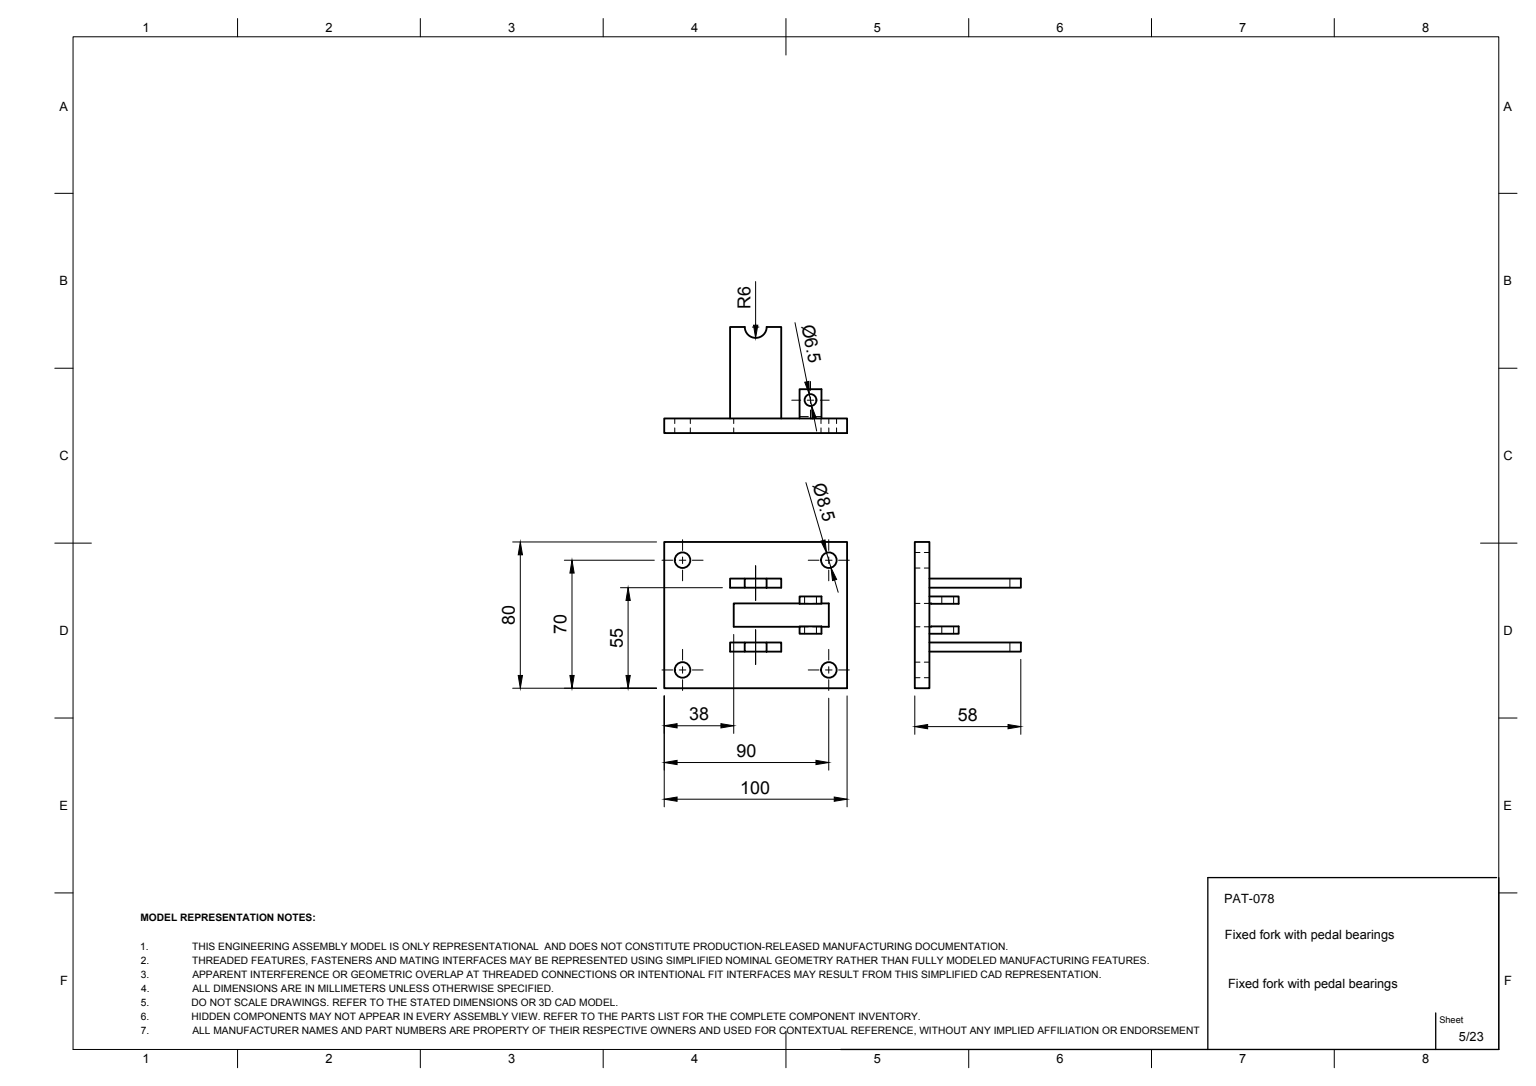
ISO-10303-21;
HEADER;
/* Generated by software containing ST-Developer
 * from STEP Tools, Inc. (www.steptools.com) 
 */

FILE_DESCRIPTION(
/* description */ ('Pedal-braked fixed caster'),
/* implementation_level */ '2;1');

FILE_NAME(
/* name */ 'Fixed fork with pedal bearings.step',
/* time_stamp */ '2026-10-28T03:26:52-07:00',
/* author */ (''),
/* organization */ (''),
/* preprocessor_version */ 'ST-DEVELOPER v20.2',
/* originating_system */ 'Autodesk Translation Framework v15.17.0.0',
/* authorisation */ '');

FILE_SCHEMA (('AUTOMOTIVE_DESIGN { 1 0 10303 214 3 1 1 }'));
ENDSEC;

DATA;
#10=MECHANICAL_DESIGN_GEOMETRIC_PRESENTATION_REPRESENTATION('',(#206),#5734);
#172=SHAPE_REPRESENTATION_RELATIONSHIP('SRR','None',#5810,#189);
#189=ADVANCED_BREP_SHAPE_REPRESENTATION('',(#230),#5714);
#206=STYLED_ITEM('',(#5984),#230);
#230=MANIFOLD_SOLID_BREP('Body1',#2987);
#253=CYLINDRICAL_SURFACE('',#3213,0.325);
#254=CYLINDRICAL_SURFACE('',#3216,0.325);
#255=CYLINDRICAL_SURFACE('',#3225,0.6);
#256=CYLINDRICAL_SURFACE('',#3228,0.6);
#257=CYLINDRICAL_SURFACE('',#3243,0.425);
#258=CYLINDRICAL_SURFACE('',#3246,0.425);
#259=CYLINDRICAL_SURFACE('',#3249,0.425);
#260=CYLINDRICAL_SURFACE('',#3252,0.425);
#295=FACE_BOUND('',#661,.T.);
#296=FACE_BOUND('',#667,.T.);
#297=FACE_BOUND('',#671,.T.);
#298=FACE_BOUND('',#675,.T.);
#299=FACE_BOUND('',#699,.T.);
#300=FACE_BOUND('',#700,.T.);
#301=FACE_BOUND('',#701,.T.);
#302=FACE_BOUND('',#702,.T.);
#303=FACE_BOUND('',#703,.T.);
#304=FACE_BOUND('',#705,.T.);
#305=FACE_BOUND('',#706,.T.);
#306=FACE_BOUND('',#707,.T.);
#307=FACE_BOUND('',#708,.T.);
#308=FACE_BOUND('',#709,.T.);
#309=FACE_BOUND('',#710,.T.);
#310=FACE_BOUND('',#711,.T.);
#340=CIRCLE('',#3210,0.325);
#341=CIRCLE('',#3214,0.325);
#342=CIRCLE('',#3215,0.325);
#343=CIRCLE('',#3217,0.325);
#344=CIRCLE('',#3226,0.6);
#345=CIRCLE('',#3227,0.6);
#346=CIRCLE('',#3229,0.6);
#347=CIRCLE('',#3230,0.6);
#348=CIRCLE('',#3244,0.425);
#349=CIRCLE('',#3245,0.425);
#350=CIRCLE('',#3247,0.425);
#351=CIRCLE('',#3248,0.425);
#352=CIRCLE('',#3250,0.425);
#353=CIRCLE('',#3251,0.425);
#354=CIRCLE('',#3253,0.425);
#355=CIRCLE('',#3254,0.425);
#476=FACE_OUTER_BOUND('',#654,.T.);
#477=FACE_OUTER_BOUND('',#655,.T.);
#478=FACE_OUTER_BOUND('',#656,.T.);
#479=FACE_OUTER_BOUND('',#657,.T.);
#480=FACE_OUTER_BOUND('',#658,.T.);
#481=FACE_OUTER_BOUND('',#659,.T.);
#482=FACE_OUTER_BOUND('',#660,.T.);
#483=FACE_OUTER_BOUND('',#662,.T.);
#484=FACE_OUTER_BOUND('',#663,.T.);
#485=FACE_OUTER_BOUND('',#664,.T.);
#486=FACE_OUTER_BOUND('',#665,.T.);
#487=FACE_OUTER_BOUND('',#666,.T.);
#488=FACE_OUTER_BOUND('',#668,.T.);
#489=FACE_OUTER_BOUND('',#669,.T.);
#490=FACE_OUTER_BOUND('',#670,.T.);
#491=FACE_OUTER_BOUND('',#672,.T.);
#492=FACE_OUTER_BOUND('',#673,.T.);
#493=FACE_OUTER_BOUND('',#674,.T.);
#494=FACE_OUTER_BOUND('',#676,.T.);
#495=FACE_OUTER_BOUND('',#677,.T.);
#496=FACE_OUTER_BOUND('',#678,.T.);
#497=FACE_OUTER_BOUND('',#679,.T.);
#498=FACE_OUTER_BOUND('',#680,.T.);
#499=FACE_OUTER_BOUND('',#681,.T.);
#500=FACE_OUTER_BOUND('',#682,.T.);
#501=FACE_OUTER_BOUND('',#683,.T.);
#502=FACE_OUTER_BOUND('',#684,.T.);
#503=FACE_OUTER_BOUND('',#685,.T.);
#504=FACE_OUTER_BOUND('',#686,.T.);
#505=FACE_OUTER_BOUND('',#687,.T.);
#506=FACE_OUTER_BOUND('',#688,.T.);
#507=FACE_OUTER_BOUND('',#689,.T.);
#508=FACE_OUTER_BOUND('',#690,.T.);
#509=FACE_OUTER_BOUND('',#691,.T.);
#510=FACE_OUTER_BOUND('',#692,.T.);
#511=FACE_OUTER_BOUND('',#693,.T.);
#512=FACE_OUTER_BOUND('',#694,.T.);
#513=FACE_OUTER_BOUND('',#695,.T.);
#514=FACE_OUTER_BOUND('',#696,.T.);
#515=FACE_OUTER_BOUND('',#697,.T.);
#516=FACE_OUTER_BOUND('',#698,.T.);
#517=FACE_OUTER_BOUND('',#704,.T.);
#654=EDGE_LOOP('',(#1940,#1941,#1942,#1943));
#655=EDGE_LOOP('',(#1944,#1945,#1946,#1947,#1948,#1949,#1950,#1951));
#656=EDGE_LOOP('',(#1952,#1953,#1954,#1955));
#657=EDGE_LOOP('',(#1956,#1957,#1958,#1959));
#658=EDGE_LOOP('',(#1960,#1961,#1962,#1963,#1964,#1965,#1966,#1967));
#659=EDGE_LOOP('',(#1968,#1969,#1970,#1971));
#660=EDGE_LOOP('',(#1972,#1973,#1974,#1975));
#661=EDGE_LOOP('',(#1976));
#662=EDGE_LOOP('',(#1977,#1978,#1979,#1980,#1981,#1982));
#663=EDGE_LOOP('',(#1983,#1984,#1985,#1986,#1987,#1988));
#664=EDGE_LOOP('',(#1989,#1990,#1991,#1992));
#665=EDGE_LOOP('',(#1993,#1994,#1995,#1996));
#666=EDGE_LOOP('',(#1997,#1998,#1999,#2000));
#667=EDGE_LOOP('',(#2001));
#668=EDGE_LOOP('',(#2002,#2003,#2004,#2005,#2006,#2007));
#669=EDGE_LOOP('',(#2008,#2009,#2010,#2011));
#670=EDGE_LOOP('',(#2012,#2013,#2014,#2015));
#671=EDGE_LOOP('',(#2016));
#672=EDGE_LOOP('',(#2017,#2018,#2019,#2020,#2021,#2022));
#673=EDGE_LOOP('',(#2023,#2024,#2025,#2026));
#674=EDGE_LOOP('',(#2027,#2028,#2029,#2030));
#675=EDGE_LOOP('',(#2031));
#676=EDGE_LOOP('',(#2032,#2033,#2034,#2035));
#677=EDGE_LOOP('',(#2036,#2037,#2038,#2039));
#678=EDGE_LOOP('',(#2040,#2041,#2042,#2043,#2044,#2045));
#679=EDGE_LOOP('',(#2046,#2047,#2048,#2049));
#680=EDGE_LOOP('',(#2050,#2051,#2052,#2053,#2054,#2055));
#681=EDGE_LOOP('',(#2056,#2057,#2058,#2059));
#682=EDGE_LOOP('',(#2060,#2061,#2062,#2063,#2064,#2065));
#683=EDGE_LOOP('',(#2066,#2067,#2068,#2069));
#684=EDGE_LOOP('',(#2070,#2071,#2072,#2073));
#685=EDGE_LOOP('',(#2074,#2075,#2076,#2077));
#686=EDGE_LOOP('',(#2078,#2079,#2080,#2081,#2082,#2083));
#687=EDGE_LOOP('',(#2084,#2085,#2086,#2087));
#688=EDGE_LOOP('',(#2088,#2089,#2090,#2091));
#689=EDGE_LOOP('',(#2092,#2093,#2094,#2095));
#690=EDGE_LOOP('',(#2096,#2097,#2098,#2099));
#691=EDGE_LOOP('',(#2100,#2101,#2102,#2103));
#692=EDGE_LOOP('',(#2104,#2105,#2106,#2107));
#693=EDGE_LOOP('',(#2108,#2109,#2110,#2111));
#694=EDGE_LOOP('',(#2112,#2113,#2114,#2115));
#695=EDGE_LOOP('',(#2116,#2117,#2118,#2119));
#696=EDGE_LOOP('',(#2120,#2121,#2122,#2123));
#697=EDGE_LOOP('',(#2124,#2125,#2126,#2127));
#698=EDGE_LOOP('',(#2128,#2129,#2130,#2131));
#699=EDGE_LOOP('',(#2132,#2133,#2134,#2135));
#700=EDGE_LOOP('',(#2136));
#701=EDGE_LOOP('',(#2137));
#702=EDGE_LOOP('',(#2138));
#703=EDGE_LOOP('',(#2139));
#704=EDGE_LOOP('',(#2140,#2141,#2142,#2143));
#705=EDGE_LOOP('',(#2144,#2145,#2146,#2147,#2148,#2149,#2150,#2151,#2152,
#2153,#2154,#2155));
#706=EDGE_LOOP('',(#2156));
#707=EDGE_LOOP('',(#2157));
#708=EDGE_LOOP('',(#2158));
#709=EDGE_LOOP('',(#2159));
#710=EDGE_LOOP('',(#2160,#2161,#2162,#2163));
#711=EDGE_LOOP('',(#2164,#2165,#2166,#2167));
#877=LINE('',#4501,#1089);
#878=LINE('',#4503,#1090);
#879=LINE('',#4505,#1091);
#880=LINE('',#4506,#1092);
#881=LINE('',#4509,#1093);
#882=LINE('',#4511,#1094);
#883=LINE('',#4513,#1095);
#884=LINE('',#4515,#1096);
#885=LINE('',#4517,#1097);
#886=LINE('',#4519,#1098);
#887=LINE('',#4520,#1099);
#888=LINE('',#4523,#1100);
#889=LINE('',#4525,#1101);
#890=LINE('',#4526,#1102);
#891=LINE('',#4530,#1103);
#892=LINE('',#4532,#1104);
#893=LINE('',#4534,#1105);
#894=LINE('',#4535,#1106);
#895=LINE('',#4538,#1107);
#896=LINE('',#4540,#1108);
#897=LINE('',#4541,#1109);
#898=LINE('',#4543,#1110);
#899=LINE('',#4545,#1111);
#900=LINE('',#4546,#1112);
#901=LINE('',#4548,#1113);
#902=LINE('',#4549,#1114);
#903=LINE('',#4552,#1115);
#904=LINE('',#4554,#1116);
#905=LINE('',#4555,#1117);
#906=LINE('',#4560,#1118);
#907=LINE('',#4562,#1119);
#908=LINE('',#4563,#1120);
#909=LINE('',#4566,#1121);
#910=LINE('',#4568,#1122);
#911=LINE('',#4570,#1123);
#912=LINE('',#4571,#1124);
#913=LINE('',#4576,#1125);
#914=LINE('',#4580,#1126);
#915=LINE('',#4584,#1127);
#916=LINE('',#4586,#1128);
#917=LINE('',#4587,#1129);
#918=LINE('',#4589,#1130);
#919=LINE('',#4590,#1131);
#920=LINE('',#4594,#1132);
#921=LINE('',#4595,#1133);
#922=LINE('',#4598,#1134);
#923=LINE('',#4600,#1135);
#924=LINE('',#4601,#1136);
#925=LINE('',#4603,#1137);
#926=LINE('',#4605,#1138);
#927=LINE('',#4611,#1139);
#928=LINE('',#4614,#1140);
#929=LINE('',#4620,#1141);
#930=LINE('',#4623,#1142);
#931=LINE('',#4626,#1143);
#932=LINE('',#4628,#1144);
#933=LINE('',#4630,#1145);
#934=LINE('',#4632,#1146);
#935=LINE('',#4633,#1147);
#936=LINE('',#4636,#1148);
#937=LINE('',#4637,#1149);
#938=LINE('',#4640,#1150);
#939=LINE('',#4642,#1151);
#940=LINE('',#4644,#1152);
#941=LINE('',#4646,#1153);
#942=LINE('',#4647,#1154);
#943=LINE('',#4650,#1155);
#944=LINE('',#4651,#1156);
#945=LINE('',#4654,#1157);
#946=LINE('',#4656,#1158);
#947=LINE('',#4658,#1159);
#948=LINE('',#4659,#1160);
#949=LINE('',#4661,#1161);
#950=LINE('',#4663,#1162);
#951=LINE('',#4664,#1163);
#952=LINE('',#4668,#1164);
#953=LINE('',#4670,#1165);
#954=LINE('',#4672,#1166);
#955=LINE('',#4673,#1167);
#956=LINE('',#4675,#1168);
#957=LINE('',#4677,#1169);
#958=LINE('',#4678,#1170);
#959=LINE('',#4684,#1171);
#960=LINE('',#4690,#1172);
#961=LINE('',#4696,#1173);
#962=LINE('',#4702,#1174);
#963=LINE('',#4707,#1175);
#964=LINE('',#4709,#1176);
#965=LINE('',#4711,#1177);
#966=LINE('',#4712,#1178);
#967=LINE('',#4715,#1179);
#968=LINE('',#4717,#1180);
#969=LINE('',#4718,#1181);
#970=LINE('',#4721,#1182);
#971=LINE('',#4723,#1183);
#972=LINE('',#4724,#1184);
#973=LINE('',#4726,#1185);
#974=LINE('',#4727,#1186);
#1089=VECTOR('',#3569,1.);
#1090=VECTOR('',#3570,1.);
#1091=VECTOR('',#3571,1.);
#1092=VECTOR('',#3572,1.);
#1093=VECTOR('',#3575,1.);
#1094=VECTOR('',#3576,1.);
#1095=VECTOR('',#3577,1.);
#1096=VECTOR('',#3578,1.);
#1097=VECTOR('',#3579,1.);
#1098=VECTOR('',#3580,1.);
#1099=VECTOR('',#3581,1.);
#1100=VECTOR('',#3584,1.);
#1101=VECTOR('',#3585,1.);
#1102=VECTOR('',#3586,1.);
#1103=VECTOR('',#3589,1.);
#1104=VECTOR('',#3590,1.);
#1105=VECTOR('',#3591,1.);
#1106=VECTOR('',#3592,1.);
#1107=VECTOR('',#3595,1.);
#1108=VECTOR('',#3596,1.);
#1109=VECTOR('',#3597,1.);
#1110=VECTOR('',#3598,1.);
#1111=VECTOR('',#3599,1.);
#1112=VECTOR('',#3600,1.);
#1113=VECTOR('',#3603,1.);
#1114=VECTOR('',#3604,1.);
#1115=VECTOR('',#3607,1.);
#1116=VECTOR('',#3608,1.);
#1117=VECTOR('',#3609,1.);
#1118=VECTOR('',#3614,1.);
#1119=VECTOR('',#3615,1.);
#1120=VECTOR('',#3616,1.);
#1121=VECTOR('',#3619,1.);
#1122=VECTOR('',#3620,1.);
#1123=VECTOR('',#3621,1.);
#1124=VECTOR('',#3622,1.);
#1125=VECTOR('',#3627,0.325);
#1126=VECTOR('',#3632,0.325);
#1127=VECTOR('',#3637,1.);
#1128=VECTOR('',#3638,1.);
#1129=VECTOR('',#3639,1.);
#1130=VECTOR('',#3642,1.);
#1131=VECTOR('',#3643,1.);
#1132=VECTOR('',#3648,1.);
#1133=VECTOR('',#3649,1.);
#1134=VECTOR('',#3652,1.);
#1135=VECTOR('',#3653,1.);
#1136=VECTOR('',#3654,1.);
#1137=VECTOR('',#3657,1.);
#1138=VECTOR('',#3660,1.);
#1139=VECTOR('',#3665,1.);
#1140=VECTOR('',#3668,1.);
#1141=VECTOR('',#3673,1.);
#1142=VECTOR('',#3676,1.);
#1143=VECTOR('',#3679,1.);
#1144=VECTOR('',#3680,1.);
#1145=VECTOR('',#3681,1.);
#1146=VECTOR('',#3682,1.);
#1147=VECTOR('',#3683,1.);
#1148=VECTOR('',#3686,1.);
#1149=VECTOR('',#3687,1.);
#1150=VECTOR('',#3690,1.);
#1151=VECTOR('',#3691,1.);
#1152=VECTOR('',#3692,1.);
#1153=VECTOR('',#3693,1.);
#1154=VECTOR('',#3694,1.);
#1155=VECTOR('',#3697,1.);
#1156=VECTOR('',#3698,1.);
#1157=VECTOR('',#3701,1.);
#1158=VECTOR('',#3702,1.);
#1159=VECTOR('',#3703,1.);
#1160=VECTOR('',#3704,1.);
#1161=VECTOR('',#3707,1.);
#1162=VECTOR('',#3710,1.);
#1163=VECTOR('',#3711,1.);
#1164=VECTOR('',#3716,1.);
#1165=VECTOR('',#3717,1.);
#1166=VECTOR('',#3718,1.);
#1167=VECTOR('',#3719,1.);
#1168=VECTOR('',#3722,1.);
#1169=VECTOR('',#3725,1.);
#1170=VECTOR('',#3726,1.);
#1171=VECTOR('',#3733,0.425);
#1172=VECTOR('',#3740,0.425);
#1173=VECTOR('',#3747,0.425);
#1174=VECTOR('',#3754,0.425);
#1175=VECTOR('',#3759,1.);
#1176=VECTOR('',#3760,1.);
#1177=VECTOR('',#3761,1.);
#1178=VECTOR('',#3762,1.);
#1179=VECTOR('',#3765,1.);
#1180=VECTOR('',#3766,1.);
#1181=VECTOR('',#3767,1.);
#1182=VECTOR('',#3770,1.);
#1183=VECTOR('',#3771,1.);
#1184=VECTOR('',#3772,1.);
#1185=VECTOR('',#3775,1.);
#1186=VECTOR('',#3776,1.);
#1301=VERTEX_POINT('',#4499);
#1302=VERTEX_POINT('',#4500);
#1303=VERTEX_POINT('',#4502);
#1304=VERTEX_POINT('',#4504);
#1305=VERTEX_POINT('',#4508);
#1306=VERTEX_POINT('',#4510);
#1307=VERTEX_POINT('',#4512);
#1308=VERTEX_POINT('',#4514);
#1309=VERTEX_POINT('',#4516);
#1310=VERTEX_POINT('',#4518);
#1311=VERTEX_POINT('',#4522);
#1312=VERTEX_POINT('',#4524);
#1313=VERTEX_POINT('',#4528);
#1314=VERTEX_POINT('',#4529);
#1315=VERTEX_POINT('',#4531);
#1316=VERTEX_POINT('',#4533);
#1317=VERTEX_POINT('',#4537);
#1318=VERTEX_POINT('',#4539);
#1319=VERTEX_POINT('',#4542);
#1320=VERTEX_POINT('',#4544);
#1321=VERTEX_POINT('',#4551);
#1322=VERTEX_POINT('',#4553);
#1323=VERTEX_POINT('',#4556);
#1324=VERTEX_POINT('',#4559);
#1325=VERTEX_POINT('',#4561);
#1326=VERTEX_POINT('',#4565);
#1327=VERTEX_POINT('',#4567);
#1328=VERTEX_POINT('',#4569);
#1329=VERTEX_POINT('',#4573);
#1330=VERTEX_POINT('',#4575);
#1331=VERTEX_POINT('',#4579);
#1332=VERTEX_POINT('',#4583);
#1333=VERTEX_POINT('',#4585);
#1334=VERTEX_POINT('',#4593);
#1335=VERTEX_POINT('',#4597);
#1336=VERTEX_POINT('',#4599);
#1337=VERTEX_POINT('',#4607);
#1338=VERTEX_POINT('',#4608);
#1339=VERTEX_POINT('',#4610);
#1340=VERTEX_POINT('',#4612);
#1341=VERTEX_POINT('',#4616);
#1342=VERTEX_POINT('',#4617);
#1343=VERTEX_POINT('',#4619);
#1344=VERTEX_POINT('',#4621);
#1345=VERTEX_POINT('',#4625);
#1346=VERTEX_POINT('',#4627);
#1347=VERTEX_POINT('',#4629);
#1348=VERTEX_POINT('',#4631);
#1349=VERTEX_POINT('',#4635);
#1350=VERTEX_POINT('',#4639);
#1351=VERTEX_POINT('',#4641);
#1352=VERTEX_POINT('',#4643);
#1353=VERTEX_POINT('',#4645);
#1354=VERTEX_POINT('',#4649);
#1355=VERTEX_POINT('',#4653);
#1356=VERTEX_POINT('',#4655);
#1357=VERTEX_POINT('',#4657);
#1358=VERTEX_POINT('',#4667);
#1359=VERTEX_POINT('',#4669);
#1360=VERTEX_POINT('',#4671);
#1361=VERTEX_POINT('',#4681);
#1362=VERTEX_POINT('',#4683);
#1363=VERTEX_POINT('',#4687);
#1364=VERTEX_POINT('',#4689);
#1365=VERTEX_POINT('',#4693);
#1366=VERTEX_POINT('',#4695);
#1367=VERTEX_POINT('',#4699);
#1368=VERTEX_POINT('',#4701);
#1369=VERTEX_POINT('',#4705);
#1370=VERTEX_POINT('',#4706);
#1371=VERTEX_POINT('',#4708);
#1372=VERTEX_POINT('',#4710);
#1373=VERTEX_POINT('',#4714);
#1374=VERTEX_POINT('',#4716);
#1375=VERTEX_POINT('',#4720);
#1376=VERTEX_POINT('',#4722);
#1560=EDGE_CURVE('',#1301,#1302,#877,.T.);
#1561=EDGE_CURVE('',#1303,#1301,#878,.T.);
#1562=EDGE_CURVE('',#1304,#1303,#879,.T.);
#1563=EDGE_CURVE('',#1304,#1302,#880,.T.);
#1564=EDGE_CURVE('',#1305,#1301,#881,.T.);
#1565=EDGE_CURVE('',#1306,#1305,#882,.T.);
#1566=EDGE_CURVE('',#1307,#1306,#883,.T.);
#1567=EDGE_CURVE('',#1308,#1307,#884,.T.);
#1568=EDGE_CURVE('',#1309,#1308,#885,.T.);
#1569=EDGE_CURVE('',#1310,#1309,#886,.T.);
#1570=EDGE_CURVE('',#1303,#1310,#887,.T.);
#1571=EDGE_CURVE('',#1311,#1308,#888,.T.);
#1572=EDGE_CURVE('',#1312,#1311,#889,.T.);
#1573=EDGE_CURVE('',#1309,#1312,#890,.T.);
#1574=EDGE_CURVE('',#1313,#1314,#891,.T.);
#1575=EDGE_CURVE('',#1313,#1315,#892,.T.);
#1576=EDGE_CURVE('',#1316,#1315,#893,.T.);
#1577=EDGE_CURVE('',#1314,#1316,#894,.T.);
#1578=EDGE_CURVE('',#1302,#1317,#895,.T.);
#1579=EDGE_CURVE('',#1318,#1304,#896,.T.);
#1580=EDGE_CURVE('',#1315,#1318,#897,.T.);
#1581=EDGE_CURVE('',#1319,#1313,#898,.T.);
#1582=EDGE_CURVE('',#1320,#1319,#899,.T.);
#1583=EDGE_CURVE('',#1320,#1317,#900,.T.);
#1584=EDGE_CURVE('',#1317,#1305,#901,.T.);
#1585=EDGE_CURVE('',#1306,#1320,#902,.T.);
#1586=EDGE_CURVE('',#1316,#1321,#903,.T.);
#1587=EDGE_CURVE('',#1321,#1322,#904,.T.);
#1588=EDGE_CURVE('',#1322,#1314,#905,.T.);
#1589=EDGE_CURVE('',#1323,#1323,#340,.T.);
#1590=EDGE_CURVE('',#1324,#1318,#906,.T.);
#1591=EDGE_CURVE('',#1325,#1324,#907,.T.);
#1592=EDGE_CURVE('',#1321,#1325,#908,.T.);
#1593=EDGE_CURVE('',#1326,#1312,#909,.T.);
#1594=EDGE_CURVE('',#1327,#1326,#910,.T.);
#1595=EDGE_CURVE('',#1328,#1327,#911,.T.);
#1596=EDGE_CURVE('',#1310,#1328,#912,.T.);
#1597=EDGE_CURVE('',#1329,#1329,#341,.T.);
#1598=EDGE_CURVE('',#1329,#1330,#913,.T.);
#1599=EDGE_CURVE('',#1330,#1330,#342,.T.);
#1600=EDGE_CURVE('',#1323,#1331,#914,.T.);
#1601=EDGE_CURVE('',#1331,#1331,#343,.T.);
#1602=EDGE_CURVE('',#1332,#1324,#915,.T.);
#1603=EDGE_CURVE('',#1332,#1333,#916,.T.);
#1604=EDGE_CURVE('',#1333,#1325,#917,.T.);
#1605=EDGE_CURVE('',#1322,#1333,#918,.T.);
#1606=EDGE_CURVE('',#1319,#1332,#919,.T.);
#1607=EDGE_CURVE('',#1311,#1334,#920,.T.);
#1608=EDGE_CURVE('',#1334,#1326,#921,.T.);
#1609=EDGE_CURVE('',#1335,#1307,#922,.T.);
#1610=EDGE_CURVE('',#1336,#1335,#923,.T.);
#1611=EDGE_CURVE('',#1336,#1334,#924,.T.);
#1612=EDGE_CURVE('',#1327,#1336,#925,.T.);
#1613=EDGE_CURVE('',#1328,#1335,#926,.T.);
#1614=EDGE_CURVE('',#1337,#1338,#344,.T.);
#1615=EDGE_CURVE('',#1339,#1337,#927,.T.);
#1616=EDGE_CURVE('',#1340,#1339,#345,.T.);
#1617=EDGE_CURVE('',#1338,#1340,#928,.T.);
#1618=EDGE_CURVE('',#1341,#1342,#346,.T.);
#1619=EDGE_CURVE('',#1343,#1341,#929,.T.);
#1620=EDGE_CURVE('',#1344,#1343,#347,.T.);
#1621=EDGE_CURVE('',#1342,#1344,#930,.T.);
#1622=EDGE_CURVE('',#1343,#1345,#931,.T.);
#1623=EDGE_CURVE('',#1345,#1346,#932,.T.);
#1624=EDGE_CURVE('',#1347,#1346,#933,.T.);
#1625=EDGE_CURVE('',#1347,#1348,#934,.T.);
#1626=EDGE_CURVE('',#1348,#1344,#935,.T.);
#1627=EDGE_CURVE('',#1349,#1341,#936,.T.);
#1628=EDGE_CURVE('',#1345,#1349,#937,.T.);
#1629=EDGE_CURVE('',#1339,#1350,#938,.T.);
#1630=EDGE_CURVE('',#1350,#1351,#939,.T.);
#1631=EDGE_CURVE('',#1352,#1351,#940,.T.);
#1632=EDGE_CURVE('',#1352,#1353,#941,.T.);
#1633=EDGE_CURVE('',#1353,#1340,#942,.T.);
#1634=EDGE_CURVE('',#1354,#1337,#943,.T.);
#1635=EDGE_CURVE('',#1350,#1354,#944,.T.);
#1636=EDGE_CURVE('',#1342,#1355,#945,.T.);
#1637=EDGE_CURVE('',#1355,#1356,#946,.T.);
#1638=EDGE_CURVE('',#1357,#1356,#947,.T.);
#1639=EDGE_CURVE('',#1357,#1349,#948,.T.);
#1640=EDGE_CURVE('',#1346,#1357,#949,.T.);
#1641=EDGE_CURVE('',#1356,#1347,#950,.T.);
#1642=EDGE_CURVE('',#1348,#1355,#951,.T.);
#1643=EDGE_CURVE('',#1338,#1358,#952,.T.);
#1644=EDGE_CURVE('',#1358,#1359,#953,.T.);
#1645=EDGE_CURVE('',#1360,#1359,#954,.T.);
#1646=EDGE_CURVE('',#1360,#1354,#955,.T.);
#1647=EDGE_CURVE('',#1351,#1360,#956,.T.);
#1648=EDGE_CURVE('',#1359,#1352,#957,.T.);
#1649=EDGE_CURVE('',#1353,#1358,#958,.T.);
#1650=EDGE_CURVE('',#1361,#1361,#348,.T.);
#1651=EDGE_CURVE('',#1361,#1362,#959,.T.);
#1652=EDGE_CURVE('',#1362,#1362,#349,.T.);
#1653=EDGE_CURVE('',#1363,#1363,#350,.T.);
#1654=EDGE_CURVE('',#1363,#1364,#960,.T.);
#1655=EDGE_CURVE('',#1364,#1364,#351,.T.);
#1656=EDGE_CURVE('',#1365,#1365,#352,.T.);
#1657=EDGE_CURVE('',#1365,#1366,#961,.T.);
#1658=EDGE_CURVE('',#1366,#1366,#353,.T.);
#1659=EDGE_CURVE('',#1367,#1367,#354,.T.);
#1660=EDGE_CURVE('',#1367,#1368,#962,.T.);
#1661=EDGE_CURVE('',#1368,#1368,#355,.T.);
#1662=EDGE_CURVE('',#1369,#1370,#963,.T.);
#1663=EDGE_CURVE('',#1370,#1371,#964,.T.);
#1664=EDGE_CURVE('',#1372,#1371,#965,.T.);
#1665=EDGE_CURVE('',#1369,#1372,#966,.T.);
#1666=EDGE_CURVE('',#1373,#1369,#967,.T.);
#1667=EDGE_CURVE('',#1374,#1372,#968,.T.);
#1668=EDGE_CURVE('',#1373,#1374,#969,.T.);
#1669=EDGE_CURVE('',#1375,#1373,#970,.T.);
#1670=EDGE_CURVE('',#1376,#1374,#971,.T.);
#1671=EDGE_CURVE('',#1375,#1376,#972,.T.);
#1672=EDGE_CURVE('',#1370,#1375,#973,.T.);
#1673=EDGE_CURVE('',#1371,#1376,#974,.T.);
#1940=ORIENTED_EDGE('',*,*,#1560,.F.);
#1941=ORIENTED_EDGE('',*,*,#1561,.F.);
#1942=ORIENTED_EDGE('',*,*,#1562,.F.);
#1943=ORIENTED_EDGE('',*,*,#1563,.T.);
#1944=ORIENTED_EDGE('',*,*,#1564,.F.);
#1945=ORIENTED_EDGE('',*,*,#1565,.F.);
#1946=ORIENTED_EDGE('',*,*,#1566,.F.);
#1947=ORIENTED_EDGE('',*,*,#1567,.F.);
#1948=ORIENTED_EDGE('',*,*,#1568,.F.);
#1949=ORIENTED_EDGE('',*,*,#1569,.F.);
#1950=ORIENTED_EDGE('',*,*,#1570,.F.);
#1951=ORIENTED_EDGE('',*,*,#1561,.T.);
#1952=ORIENTED_EDGE('',*,*,#1571,.F.);
#1953=ORIENTED_EDGE('',*,*,#1572,.F.);
#1954=ORIENTED_EDGE('',*,*,#1573,.F.);
#1955=ORIENTED_EDGE('',*,*,#1568,.T.);
#1956=ORIENTED_EDGE('',*,*,#1574,.F.);
#1957=ORIENTED_EDGE('',*,*,#1575,.T.);
#1958=ORIENTED_EDGE('',*,*,#1576,.F.);
#1959=ORIENTED_EDGE('',*,*,#1577,.F.);
#1960=ORIENTED_EDGE('',*,*,#1578,.F.);
#1961=ORIENTED_EDGE('',*,*,#1563,.F.);
#1962=ORIENTED_EDGE('',*,*,#1579,.F.);
#1963=ORIENTED_EDGE('',*,*,#1580,.F.);
#1964=ORIENTED_EDGE('',*,*,#1575,.F.);
#1965=ORIENTED_EDGE('',*,*,#1581,.F.);
#1966=ORIENTED_EDGE('',*,*,#1582,.F.);
#1967=ORIENTED_EDGE('',*,*,#1583,.T.);
#1968=ORIENTED_EDGE('',*,*,#1584,.F.);
#1969=ORIENTED_EDGE('',*,*,#1583,.F.);
#1970=ORIENTED_EDGE('',*,*,#1585,.F.);
#1971=ORIENTED_EDGE('',*,*,#1565,.T.);
#1972=ORIENTED_EDGE('',*,*,#1577,.T.);
#1973=ORIENTED_EDGE('',*,*,#1586,.T.);
#1974=ORIENTED_EDGE('',*,*,#1587,.T.);
#1975=ORIENTED_EDGE('',*,*,#1588,.T.);
#1976=ORIENTED_EDGE('',*,*,#1589,.T.);
#1977=ORIENTED_EDGE('',*,*,#1576,.T.);
#1978=ORIENTED_EDGE('',*,*,#1580,.T.);
#1979=ORIENTED_EDGE('',*,*,#1590,.F.);
#1980=ORIENTED_EDGE('',*,*,#1591,.F.);
#1981=ORIENTED_EDGE('',*,*,#1592,.F.);
#1982=ORIENTED_EDGE('',*,*,#1586,.F.);
#1983=ORIENTED_EDGE('',*,*,#1569,.T.);
#1984=ORIENTED_EDGE('',*,*,#1573,.T.);
#1985=ORIENTED_EDGE('',*,*,#1593,.F.);
#1986=ORIENTED_EDGE('',*,*,#1594,.F.);
#1987=ORIENTED_EDGE('',*,*,#1595,.F.);
#1988=ORIENTED_EDGE('',*,*,#1596,.F.);
#1989=ORIENTED_EDGE('',*,*,#1597,.F.);
#1990=ORIENTED_EDGE('',*,*,#1598,.T.);
#1991=ORIENTED_EDGE('',*,*,#1599,.F.);
#1992=ORIENTED_EDGE('',*,*,#1598,.F.);
#1993=ORIENTED_EDGE('',*,*,#1589,.F.);
#1994=ORIENTED_EDGE('',*,*,#1600,.T.);
#1995=ORIENTED_EDGE('',*,*,#1601,.F.);
#1996=ORIENTED_EDGE('',*,*,#1600,.F.);
#1997=ORIENTED_EDGE('',*,*,#1602,.F.);
#1998=ORIENTED_EDGE('',*,*,#1603,.T.);
#1999=ORIENTED_EDGE('',*,*,#1604,.T.);
#2000=ORIENTED_EDGE('',*,*,#1591,.T.);
#2001=ORIENTED_EDGE('',*,*,#1601,.T.);
#2002=ORIENTED_EDGE('',*,*,#1574,.T.);
#2003=ORIENTED_EDGE('',*,*,#1588,.F.);
#2004=ORIENTED_EDGE('',*,*,#1605,.T.);
#2005=ORIENTED_EDGE('',*,*,#1603,.F.);
#2006=ORIENTED_EDGE('',*,*,#1606,.F.);
#2007=ORIENTED_EDGE('',*,*,#1581,.T.);
#2008=ORIENTED_EDGE('',*,*,#1587,.F.);
#2009=ORIENTED_EDGE('',*,*,#1592,.T.);
#2010=ORIENTED_EDGE('',*,*,#1604,.F.);
#2011=ORIENTED_EDGE('',*,*,#1605,.F.);
#2012=ORIENTED_EDGE('',*,*,#1572,.T.);
#2013=ORIENTED_EDGE('',*,*,#1607,.T.);
#2014=ORIENTED_EDGE('',*,*,#1608,.T.);
#2015=ORIENTED_EDGE('',*,*,#1593,.T.);
#2016=ORIENTED_EDGE('',*,*,#1599,.T.);
#2017=ORIENTED_EDGE('',*,*,#1567,.T.);
#2018=ORIENTED_EDGE('',*,*,#1609,.F.);
#2019=ORIENTED_EDGE('',*,*,#1610,.F.);
#2020=ORIENTED_EDGE('',*,*,#1611,.T.);
#2021=ORIENTED_EDGE('',*,*,#1607,.F.);
#2022=ORIENTED_EDGE('',*,*,#1571,.T.);
#2023=ORIENTED_EDGE('',*,*,#1612,.F.);
#2024=ORIENTED_EDGE('',*,*,#1594,.T.);
#2025=ORIENTED_EDGE('',*,*,#1608,.F.);
#2026=ORIENTED_EDGE('',*,*,#1611,.F.);
#2027=ORIENTED_EDGE('',*,*,#1613,.F.);
#2028=ORIENTED_EDGE('',*,*,#1595,.T.);
#2029=ORIENTED_EDGE('',*,*,#1612,.T.);
#2030=ORIENTED_EDGE('',*,*,#1610,.T.);
#2031=ORIENTED_EDGE('',*,*,#1597,.T.);
#2032=ORIENTED_EDGE('',*,*,#1614,.F.);
#2033=ORIENTED_EDGE('',*,*,#1615,.F.);
#2034=ORIENTED_EDGE('',*,*,#1616,.F.);
#2035=ORIENTED_EDGE('',*,*,#1617,.F.);
#2036=ORIENTED_EDGE('',*,*,#1618,.F.);
#2037=ORIENTED_EDGE('',*,*,#1619,.F.);
#2038=ORIENTED_EDGE('',*,*,#1620,.F.);
#2039=ORIENTED_EDGE('',*,*,#1621,.F.);
#2040=ORIENTED_EDGE('',*,*,#1620,.T.);
#2041=ORIENTED_EDGE('',*,*,#1622,.T.);
#2042=ORIENTED_EDGE('',*,*,#1623,.T.);
#2043=ORIENTED_EDGE('',*,*,#1624,.F.);
#2044=ORIENTED_EDGE('',*,*,#1625,.T.);
#2045=ORIENTED_EDGE('',*,*,#1626,.T.);
#2046=ORIENTED_EDGE('',*,*,#1619,.T.);
#2047=ORIENTED_EDGE('',*,*,#1627,.F.);
#2048=ORIENTED_EDGE('',*,*,#1628,.F.);
#2049=ORIENTED_EDGE('',*,*,#1622,.F.);
#2050=ORIENTED_EDGE('',*,*,#1616,.T.);
#2051=ORIENTED_EDGE('',*,*,#1629,.T.);
#2052=ORIENTED_EDGE('',*,*,#1630,.T.);
#2053=ORIENTED_EDGE('',*,*,#1631,.F.);
#2054=ORIENTED_EDGE('',*,*,#1632,.T.);
#2055=ORIENTED_EDGE('',*,*,#1633,.T.);
#2056=ORIENTED_EDGE('',*,*,#1615,.T.);
#2057=ORIENTED_EDGE('',*,*,#1634,.F.);
#2058=ORIENTED_EDGE('',*,*,#1635,.F.);
#2059=ORIENTED_EDGE('',*,*,#1629,.F.);
#2060=ORIENTED_EDGE('',*,*,#1618,.T.);
#2061=ORIENTED_EDGE('',*,*,#1636,.T.);
#2062=ORIENTED_EDGE('',*,*,#1637,.T.);
#2063=ORIENTED_EDGE('',*,*,#1638,.F.);
#2064=ORIENTED_EDGE('',*,*,#1639,.T.);
#2065=ORIENTED_EDGE('',*,*,#1627,.T.);
#2066=ORIENTED_EDGE('',*,*,#1640,.F.);
#2067=ORIENTED_EDGE('',*,*,#1623,.F.);
#2068=ORIENTED_EDGE('',*,*,#1628,.T.);
#2069=ORIENTED_EDGE('',*,*,#1639,.F.);
#2070=ORIENTED_EDGE('',*,*,#1641,.F.);
#2071=ORIENTED_EDGE('',*,*,#1637,.F.);
#2072=ORIENTED_EDGE('',*,*,#1642,.F.);
#2073=ORIENTED_EDGE('',*,*,#1625,.F.);
#2074=ORIENTED_EDGE('',*,*,#1621,.T.);
#2075=ORIENTED_EDGE('',*,*,#1626,.F.);
#2076=ORIENTED_EDGE('',*,*,#1642,.T.);
#2077=ORIENTED_EDGE('',*,*,#1636,.F.);
#2078=ORIENTED_EDGE('',*,*,#1614,.T.);
#2079=ORIENTED_EDGE('',*,*,#1643,.T.);
#2080=ORIENTED_EDGE('',*,*,#1644,.T.);
#2081=ORIENTED_EDGE('',*,*,#1645,.F.);
#2082=ORIENTED_EDGE('',*,*,#1646,.T.);
#2083=ORIENTED_EDGE('',*,*,#1634,.T.);
#2084=ORIENTED_EDGE('',*,*,#1647,.F.);
#2085=ORIENTED_EDGE('',*,*,#1630,.F.);
#2086=ORIENTED_EDGE('',*,*,#1635,.T.);
#2087=ORIENTED_EDGE('',*,*,#1646,.F.);
#2088=ORIENTED_EDGE('',*,*,#1648,.F.);
#2089=ORIENTED_EDGE('',*,*,#1644,.F.);
#2090=ORIENTED_EDGE('',*,*,#1649,.F.);
#2091=ORIENTED_EDGE('',*,*,#1632,.F.);
#2092=ORIENTED_EDGE('',*,*,#1617,.T.);
#2093=ORIENTED_EDGE('',*,*,#1633,.F.);
#2094=ORIENTED_EDGE('',*,*,#1649,.T.);
#2095=ORIENTED_EDGE('',*,*,#1643,.F.);
#2096=ORIENTED_EDGE('',*,*,#1650,.F.);
#2097=ORIENTED_EDGE('',*,*,#1651,.T.);
#2098=ORIENTED_EDGE('',*,*,#1652,.F.);
#2099=ORIENTED_EDGE('',*,*,#1651,.F.);
#2100=ORIENTED_EDGE('',*,*,#1653,.F.);
#2101=ORIENTED_EDGE('',*,*,#1654,.T.);
#2102=ORIENTED_EDGE('',*,*,#1655,.F.);
#2103=ORIENTED_EDGE('',*,*,#1654,.F.);
#2104=ORIENTED_EDGE('',*,*,#1656,.F.);
#2105=ORIENTED_EDGE('',*,*,#1657,.T.);
#2106=ORIENTED_EDGE('',*,*,#1658,.F.);
#2107=ORIENTED_EDGE('',*,*,#1657,.F.);
#2108=ORIENTED_EDGE('',*,*,#1659,.F.);
#2109=ORIENTED_EDGE('',*,*,#1660,.T.);
#2110=ORIENTED_EDGE('',*,*,#1661,.F.);
#2111=ORIENTED_EDGE('',*,*,#1660,.F.);
#2112=ORIENTED_EDGE('',*,*,#1662,.T.);
#2113=ORIENTED_EDGE('',*,*,#1663,.T.);
#2114=ORIENTED_EDGE('',*,*,#1664,.F.);
#2115=ORIENTED_EDGE('',*,*,#1665,.F.);
#2116=ORIENTED_EDGE('',*,*,#1666,.T.);
#2117=ORIENTED_EDGE('',*,*,#1665,.T.);
#2118=ORIENTED_EDGE('',*,*,#1667,.F.);
#2119=ORIENTED_EDGE('',*,*,#1668,.F.);
#2120=ORIENTED_EDGE('',*,*,#1669,.T.);
#2121=ORIENTED_EDGE('',*,*,#1668,.T.);
#2122=ORIENTED_EDGE('',*,*,#1670,.F.);
#2123=ORIENTED_EDGE('',*,*,#1671,.F.);
#2124=ORIENTED_EDGE('',*,*,#1672,.T.);
#2125=ORIENTED_EDGE('',*,*,#1671,.T.);
#2126=ORIENTED_EDGE('',*,*,#1673,.F.);
#2127=ORIENTED_EDGE('',*,*,#1663,.F.);
#2128=ORIENTED_EDGE('',*,*,#1673,.T.);
#2129=ORIENTED_EDGE('',*,*,#1670,.T.);
#2130=ORIENTED_EDGE('',*,*,#1667,.T.);
#2131=ORIENTED_EDGE('',*,*,#1664,.T.);
#2132=ORIENTED_EDGE('',*,*,#1578,.T.);
#2133=ORIENTED_EDGE('',*,*,#1584,.T.);
#2134=ORIENTED_EDGE('',*,*,#1564,.T.);
#2135=ORIENTED_EDGE('',*,*,#1560,.T.);
#2136=ORIENTED_EDGE('',*,*,#1652,.T.);
#2137=ORIENTED_EDGE('',*,*,#1655,.T.);
#2138=ORIENTED_EDGE('',*,*,#1658,.T.);
#2139=ORIENTED_EDGE('',*,*,#1661,.T.);
#2140=ORIENTED_EDGE('',*,*,#1672,.F.);
#2141=ORIENTED_EDGE('',*,*,#1662,.F.);
#2142=ORIENTED_EDGE('',*,*,#1666,.F.);
#2143=ORIENTED_EDGE('',*,*,#1669,.F.);
#2144=ORIENTED_EDGE('',*,*,#1582,.T.);
#2145=ORIENTED_EDGE('',*,*,#1606,.T.);
#2146=ORIENTED_EDGE('',*,*,#1602,.T.);
#2147=ORIENTED_EDGE('',*,*,#1590,.T.);
#2148=ORIENTED_EDGE('',*,*,#1579,.T.);
#2149=ORIENTED_EDGE('',*,*,#1562,.T.);
#2150=ORIENTED_EDGE('',*,*,#1570,.T.);
#2151=ORIENTED_EDGE('',*,*,#1596,.T.);
#2152=ORIENTED_EDGE('',*,*,#1613,.T.);
#2153=ORIENTED_EDGE('',*,*,#1609,.T.);
#2154=ORIENTED_EDGE('',*,*,#1566,.T.);
#2155=ORIENTED_EDGE('',*,*,#1585,.T.);
#2156=ORIENTED_EDGE('',*,*,#1659,.T.);
#2157=ORIENTED_EDGE('',*,*,#1656,.T.);
#2158=ORIENTED_EDGE('',*,*,#1653,.T.);
#2159=ORIENTED_EDGE('',*,*,#1650,.T.);
#2160=ORIENTED_EDGE('',*,*,#1647,.T.);
#2161=ORIENTED_EDGE('',*,*,#1645,.T.);
#2162=ORIENTED_EDGE('',*,*,#1648,.T.);
#2163=ORIENTED_EDGE('',*,*,#1631,.T.);
#2164=ORIENTED_EDGE('',*,*,#1640,.T.);
#2165=ORIENTED_EDGE('',*,*,#1638,.T.);
#2166=ORIENTED_EDGE('',*,*,#1641,.T.);
#2167=ORIENTED_EDGE('',*,*,#1624,.T.);
#2700=PLANE('',#3203);
#2701=PLANE('',#3204);
#2702=PLANE('',#3205);
#2703=PLANE('',#3206);
#2704=PLANE('',#3207);
#2705=PLANE('',#3208);
#2706=PLANE('',#3209);
#2707=PLANE('',#3211);
#2708=PLANE('',#3212);
#2709=PLANE('',#3218);
#2710=PLANE('',#3219);
#2711=PLANE('',#3220);
#2712=PLANE('',#3221);
#2713=PLANE('',#3222);
#2714=PLANE('',#3223);
#2715=PLANE('',#3224);
#2716=PLANE('',#3231);
#2717=PLANE('',#3232);
#2718=PLANE('',#3233);
#2719=PLANE('',#3234);
#2720=PLANE('',#3235);
#2721=PLANE('',#3236);
#2722=PLANE('',#3237);
#2723=PLANE('',#3238);
#2724=PLANE('',#3239);
#2725=PLANE('',#3240);
#2726=PLANE('',#3241);
#2727=PLANE('',#3242);
#2728=PLANE('',#3255);
#2729=PLANE('',#3256);
#2730=PLANE('',#3257);
#2731=PLANE('',#3258);
#2732=PLANE('',#3259);
#2733=PLANE('',#3260);
#2809=ADVANCED_FACE('',(#476),#2700,.F.);
#2810=ADVANCED_FACE('',(#477),#2701,.F.);
#2811=ADVANCED_FACE('',(#478),#2702,.T.);
#2812=ADVANCED_FACE('',(#479),#2703,.T.);
#2813=ADVANCED_FACE('',(#480),#2704,.F.);
#2814=ADVANCED_FACE('',(#481),#2705,.F.);
#2815=ADVANCED_FACE('',(#482,#295),#2706,.F.);
#2816=ADVANCED_FACE('',(#483),#2707,.T.);
#2817=ADVANCED_FACE('',(#484),#2708,.T.);
#2818=ADVANCED_FACE('',(#485),#253,.F.);
#2819=ADVANCED_FACE('',(#486),#254,.F.);
#2820=ADVANCED_FACE('',(#487,#296),#2709,.T.);
#2821=ADVANCED_FACE('',(#488),#2710,.T.);
#2822=ADVANCED_FACE('',(#489),#2711,.T.);
#2823=ADVANCED_FACE('',(#490,#297),#2712,.T.);
#2824=ADVANCED_FACE('',(#491),#2713,.T.);
#2825=ADVANCED_FACE('',(#492),#2714,.T.);
#2826=ADVANCED_FACE('',(#493,#298),#2715,.F.);
#2827=ADVANCED_FACE('',(#494),#255,.F.);
#2828=ADVANCED_FACE('',(#495),#256,.F.);
#2829=ADVANCED_FACE('',(#496),#2716,.F.);
#2830=ADVANCED_FACE('',(#497),#2717,.T.);
#2831=ADVANCED_FACE('',(#498),#2718,.F.);
#2832=ADVANCED_FACE('',(#499),#2719,.T.);
#2833=ADVANCED_FACE('',(#500),#2720,.T.);
#2834=ADVANCED_FACE('',(#501),#2721,.T.);
#2835=ADVANCED_FACE('',(#502),#2722,.T.);
#2836=ADVANCED_FACE('',(#503),#2723,.T.);
#2837=ADVANCED_FACE('',(#504),#2724,.T.);
#2838=ADVANCED_FACE('',(#505),#2725,.T.);
#2839=ADVANCED_FACE('',(#506),#2726,.T.);
#2840=ADVANCED_FACE('',(#507),#2727,.T.);
#2841=ADVANCED_FACE('',(#508),#257,.F.);
#2842=ADVANCED_FACE('',(#509),#258,.F.);
#2843=ADVANCED_FACE('',(#510),#259,.F.);
#2844=ADVANCED_FACE('',(#511),#260,.F.);
#2845=ADVANCED_FACE('',(#512),#2728,.T.);
#2846=ADVANCED_FACE('',(#513),#2729,.T.);
#2847=ADVANCED_FACE('',(#514),#2730,.T.);
#2848=ADVANCED_FACE('',(#515),#2731,.T.);
#2849=ADVANCED_FACE('',(#516,#299,#300,#301,#302,#303),#2732,.T.);
#2850=ADVANCED_FACE('',(#517,#304,#305,#306,#307,#308,#309,#310),#2733,
 .F.);
#2987=CLOSED_SHELL('',(#2809,#2810,#2811,#2812,#2813,#2814,#2815,#2816,
#2817,#2818,#2819,#2820,#2821,#2822,#2823,#2824,#2825,#2826,#2827,#2828,
#2829,#2830,#2831,#2832,#2833,#2834,#2835,#2836,#2837,#2838,#2839,#2840,
#2841,#2842,#2843,#2844,#2845,#2846,#2847,#2848,#2849,#2850));
#3202=AXIS2_PLACEMENT_3D('',#4497,#3565,#3566);
#3203=AXIS2_PLACEMENT_3D('',#4498,#3567,#3568);
#3204=AXIS2_PLACEMENT_3D('',#4507,#3573,#3574);
#3205=AXIS2_PLACEMENT_3D('',#4521,#3582,#3583);
#3206=AXIS2_PLACEMENT_3D('',#4527,#3587,#3588);
#3207=AXIS2_PLACEMENT_3D('',#4536,#3593,#3594);
#3208=AXIS2_PLACEMENT_3D('',#4547,#3601,#3602);
#3209=AXIS2_PLACEMENT_3D('',#4550,#3605,#3606);
#3210=AXIS2_PLACEMENT_3D('',#4557,#3610,#3611);
#3211=AXIS2_PLACEMENT_3D('',#4558,#3612,#3613);
#3212=AXIS2_PLACEMENT_3D('',#4564,#3617,#3618);
#3213=AXIS2_PLACEMENT_3D('',#4572,#3623,#3624);
#3214=AXIS2_PLACEMENT_3D('',#4574,#3625,#3626);
#3215=AXIS2_PLACEMENT_3D('',#4577,#3628,#3629);
#3216=AXIS2_PLACEMENT_3D('',#4578,#3630,#3631);
#3217=AXIS2_PLACEMENT_3D('',#4581,#3633,#3634);
#3218=AXIS2_PLACEMENT_3D('',#4582,#3635,#3636);
#3219=AXIS2_PLACEMENT_3D('',#4588,#3640,#3641);
#3220=AXIS2_PLACEMENT_3D('',#4591,#3644,#3645);
#3221=AXIS2_PLACEMENT_3D('',#4592,#3646,#3647);
#3222=AXIS2_PLACEMENT_3D('',#4596,#3650,#3651);
#3223=AXIS2_PLACEMENT_3D('',#4602,#3655,#3656);
#3224=AXIS2_PLACEMENT_3D('',#4604,#3658,#3659);
#3225=AXIS2_PLACEMENT_3D('',#4606,#3661,#3662);
#3226=AXIS2_PLACEMENT_3D('',#4609,#3663,#3664);
#3227=AXIS2_PLACEMENT_3D('',#4613,#3666,#3667);
#3228=AXIS2_PLACEMENT_3D('',#4615,#3669,#3670);
#3229=AXIS2_PLACEMENT_3D('',#4618,#3671,#3672);
#3230=AXIS2_PLACEMENT_3D('',#4622,#3674,#3675);
#3231=AXIS2_PLACEMENT_3D('',#4624,#3677,#3678);
#3232=AXIS2_PLACEMENT_3D('',#4634,#3684,#3685);
#3233=AXIS2_PLACEMENT_3D('',#4638,#3688,#3689);
#3234=AXIS2_PLACEMENT_3D('',#4648,#3695,#3696);
#3235=AXIS2_PLACEMENT_3D('',#4652,#3699,#3700);
#3236=AXIS2_PLACEMENT_3D('',#4660,#3705,#3706);
#3237=AXIS2_PLACEMENT_3D('',#4662,#3708,#3709);
#3238=AXIS2_PLACEMENT_3D('',#4665,#3712,#3713);
#3239=AXIS2_PLACEMENT_3D('',#4666,#3714,#3715);
#3240=AXIS2_PLACEMENT_3D('',#4674,#3720,#3721);
#3241=AXIS2_PLACEMENT_3D('',#4676,#3723,#3724);
#3242=AXIS2_PLACEMENT_3D('',#4679,#3727,#3728);
#3243=AXIS2_PLACEMENT_3D('',#4680,#3729,#3730);
#3244=AXIS2_PLACEMENT_3D('',#4682,#3731,#3732);
#3245=AXIS2_PLACEMENT_3D('',#4685,#3734,#3735);
#3246=AXIS2_PLACEMENT_3D('',#4686,#3736,#3737);
#3247=AXIS2_PLACEMENT_3D('',#4688,#3738,#3739);
#3248=AXIS2_PLACEMENT_3D('',#4691,#3741,#3742);
#3249=AXIS2_PLACEMENT_3D('',#4692,#3743,#3744);
#3250=AXIS2_PLACEMENT_3D('',#4694,#3745,#3746);
#3251=AXIS2_PLACEMENT_3D('',#4697,#3748,#3749);
#3252=AXIS2_PLACEMENT_3D('',#4698,#3750,#3751);
#3253=AXIS2_PLACEMENT_3D('',#4700,#3752,#3753);
#3254=AXIS2_PLACEMENT_3D('',#4703,#3755,#3756);
#3255=AXIS2_PLACEMENT_3D('',#4704,#3757,#3758);
#3256=AXIS2_PLACEMENT_3D('',#4713,#3763,#3764);
#3257=AXIS2_PLACEMENT_3D('',#4719,#3768,#3769);
#3258=AXIS2_PLACEMENT_3D('',#4725,#3773,#3774);
#3259=AXIS2_PLACEMENT_3D('',#4728,#3777,#3778);
#3260=AXIS2_PLACEMENT_3D('',#4729,#3779,#3780);
#3565=DIRECTION('axis',(0.,0.,1.));
#3566=DIRECTION('refdir',(1.,0.,0.));
#3567=DIRECTION('center_axis',(-1.,0.,0.));
#3568=DIRECTION('ref_axis',(0.,-1.,0.));
#3569=DIRECTION('',(0.,1.,0.));
#3570=DIRECTION('',(0.,0.,1.));
#3571=DIRECTION('',(0.,-1.,0.));
#3572=DIRECTION('',(0.,0.,1.));
#3573=DIRECTION('center_axis',(0.,-1.,0.));
#3574=DIRECTION('ref_axis',(1.,0.,0.));
#3575=DIRECTION('',(-1.,0.,0.));
#3576=DIRECTION('',(0.,0.,1.));
#3577=DIRECTION('',(1.,0.,0.));
#3578=DIRECTION('',(0.,0.,1.));
#3579=DIRECTION('',(1.,0.,0.));
#3580=DIRECTION('',(0.,0.,-1.));
#3581=DIRECTION('',(1.,0.,0.));
#3582=DIRECTION('center_axis',(0.,0.,1.));
#3583=DIRECTION('ref_axis',(1.,0.,0.));
#3584=DIRECTION('',(0.,-1.,0.));
#3585=DIRECTION('',(1.,0.,0.));
#3586=DIRECTION('',(0.,1.,0.));
#3587=DIRECTION('center_axis',(0.,0.,1.));
#3588=DIRECTION('ref_axis',(1.,0.,0.));
#3589=DIRECTION('',(0.,-1.,0.));
#3590=DIRECTION('',(-1.,0.,0.));
#3591=DIRECTION('',(0.,1.,0.));
#3592=DIRECTION('',(-1.,0.,0.));
#3593=DIRECTION('center_axis',(0.,1.,0.));
#3594=DIRECTION('ref_axis',(-1.,0.,0.));
#3595=DIRECTION('',(1.,0.,0.));
#3596=DIRECTION('',(-1.,0.,0.));
#3597=DIRECTION('',(0.,0.,1.));
#3598=DIRECTION('',(0.,0.,-1.));
#3599=DIRECTION('',(-1.,0.,0.));
#3600=DIRECTION('',(0.,0.,1.));
#3601=DIRECTION('center_axis',(1.,0.,0.));
#3602=DIRECTION('ref_axis',(0.,1.,0.));
#3603=DIRECTION('',(0.,-1.,0.));
#3604=DIRECTION('',(0.,1.,0.));
#3605=DIRECTION('center_axis',(0.,1.,0.));
#3606=DIRECTION('ref_axis',(1.,0.,0.));
#3607=DIRECTION('',(0.,0.,-1.));
#3608=DIRECTION('',(1.,0.,0.));
#3609=DIRECTION('',(0.,0.,1.));
#3610=DIRECTION('center_axis',(0.,1.,0.));
#3611=DIRECTION('ref_axis',(1.,0.,0.));
#3612=DIRECTION('center_axis',(-1.,0.,0.));
#3613=DIRECTION('ref_axis',(0.,0.,1.));
#3614=DIRECTION('',(0.,-1.,0.));
#3615=DIRECTION('',(0.,0.,1.));
#3616=DIRECTION('',(0.,1.,0.));
#3617=DIRECTION('center_axis',(-1.,0.,0.));
#3618=DIRECTION('ref_axis',(0.,0.,1.));
#3619=DIRECTION('',(0.,0.,1.));
#3620=DIRECTION('',(0.,1.,0.));
#3621=DIRECTION('',(0.,0.,-1.));
#3622=DIRECTION('',(0.,-1.,0.));
#3623=DIRECTION('center_axis',(0.,1.,0.));
#3624=DIRECTION('ref_axis',(1.,0.,0.));
#3625=DIRECTION('center_axis',(0.,1.,0.));
#3626=DIRECTION('ref_axis',(1.,0.,0.));
#3627=DIRECTION('',(0.,1.,0.));
#3628=DIRECTION('center_axis',(0.,-1.,0.));
#3629=DIRECTION('ref_axis',(1.,0.,0.));
#3630=DIRECTION('center_axis',(0.,1.,0.));
#3631=DIRECTION('ref_axis',(1.,0.,0.));
#3632=DIRECTION('',(0.,1.,0.));
#3633=DIRECTION('center_axis',(0.,-1.,0.));
#3634=DIRECTION('ref_axis',(1.,0.,0.));
#3635=DIRECTION('center_axis',(0.,1.,0.));
#3636=DIRECTION('ref_axis',(0.,0.,1.));
#3637=DIRECTION('',(-1.,0.,0.));
#3638=DIRECTION('',(0.,0.,-1.));
#3639=DIRECTION('',(-1.,0.,0.));
#3640=DIRECTION('center_axis',(1.,0.,0.));
#3641=DIRECTION('ref_axis',(0.,0.,-1.));
#3642=DIRECTION('',(0.,1.,0.));
#3643=DIRECTION('',(0.,1.,0.));
#3644=DIRECTION('center_axis',(0.,0.,-1.));
#3645=DIRECTION('ref_axis',(-1.,0.,0.));
#3646=DIRECTION('center_axis',(0.,1.,0.));
#3647=DIRECTION('ref_axis',(0.,0.,1.));
#3648=DIRECTION('',(0.,0.,-1.));
#3649=DIRECTION('',(-1.,0.,0.));
#3650=DIRECTION('center_axis',(1.,0.,0.));
#3651=DIRECTION('ref_axis',(0.,0.,-1.));
#3652=DIRECTION('',(0.,1.,0.));
#3653=DIRECTION('',(0.,0.,1.));
#3654=DIRECTION('',(0.,1.,0.));
#3655=DIRECTION('center_axis',(0.,0.,-1.));
#3656=DIRECTION('ref_axis',(-1.,0.,0.));
#3657=DIRECTION('',(1.,0.,0.));
#3658=DIRECTION('center_axis',(0.,1.,0.));
#3659=DIRECTION('ref_axis',(1.,0.,0.));
#3660=DIRECTION('',(1.,0.,0.));
#3661=DIRECTION('center_axis',(0.,1.,0.));
#3662=DIRECTION('ref_axis',(1.,0.,0.));
#3663=DIRECTION('center_axis',(0.,-1.,0.));
#3664=DIRECTION('ref_axis',(1.,0.,0.));
#3665=DIRECTION('',(0.,1.,0.));
#3666=DIRECTION('center_axis',(0.,1.,0.));
#3667=DIRECTION('ref_axis',(1.,0.,0.));
#3668=DIRECTION('',(0.,-1.,0.));
#3669=DIRECTION('center_axis',(0.,1.,0.));
#3670=DIRECTION('ref_axis',(1.,0.,0.));
#3671=DIRECTION('center_axis',(0.,-1.,0.));
#3672=DIRECTION('ref_axis',(1.,0.,0.));
#3673=DIRECTION('',(0.,1.,0.));
#3674=DIRECTION('center_axis',(0.,1.,0.));
#3675=DIRECTION('ref_axis',(1.,0.,0.));
#3676=DIRECTION('',(0.,-1.,0.));
#3677=DIRECTION('center_axis',(0.,1.,0.));
#3678=DIRECTION('ref_axis',(1.,0.,0.));
#3679=DIRECTION('',(1.,0.,0.));
#3680=DIRECTION('',(0.,0.,1.));
#3681=DIRECTION('',(1.,0.,0.));
#3682=DIRECTION('',(0.,0.,-1.));
#3683=DIRECTION('',(1.,0.,0.));
#3684=DIRECTION('center_axis',(0.,0.,-1.));
#3685=DIRECTION('ref_axis',(-1.,0.,0.));
#3686=DIRECTION('',(-1.,0.,0.));
#3687=DIRECTION('',(0.,1.,0.));
#3688=DIRECTION('center_axis',(0.,1.,0.));
#3689=DIRECTION('ref_axis',(1.,0.,0.));
#3690=DIRECTION('',(1.,0.,0.));
#3691=DIRECTION('',(0.,0.,1.));
#3692=DIRECTION('',(1.,0.,0.));
#3693=DIRECTION('',(0.,0.,-1.));
#3694=DIRECTION('',(1.,0.,0.));
#3695=DIRECTION('center_axis',(0.,0.,-1.));
#3696=DIRECTION('ref_axis',(-1.,0.,0.));
#3697=DIRECTION('',(-1.,0.,0.));
#3698=DIRECTION('',(0.,1.,0.));
#3699=DIRECTION('center_axis',(0.,1.,0.));
#3700=DIRECTION('ref_axis',(0.,0.,1.));
#3701=DIRECTION('',(-1.,0.,0.));
#3702=DIRECTION('',(0.,0.,1.));
#3703=DIRECTION('',(-1.,0.,0.));
#3704=DIRECTION('',(0.,0.,-1.));
#3705=DIRECTION('center_axis',(1.,0.,0.));
#3706=DIRECTION('ref_axis',(0.,0.,-1.));
#3707=DIRECTION('',(0.,1.,0.));
#3708=DIRECTION('center_axis',(-1.,0.,0.));
#3709=DIRECTION('ref_axis',(0.,0.,1.));
#3710=DIRECTION('',(0.,-1.,0.));
#3711=DIRECTION('',(0.,1.,0.));
#3712=DIRECTION('center_axis',(0.,0.,-1.));
#3713=DIRECTION('ref_axis',(-1.,0.,0.));
#3714=DIRECTION('center_axis',(0.,1.,0.));
#3715=DIRECTION('ref_axis',(0.,0.,1.));
#3716=DIRECTION('',(-1.,0.,0.));
#3717=DIRECTION('',(0.,0.,1.));
#3718=DIRECTION('',(-1.,0.,0.));
#3719=DIRECTION('',(0.,0.,-1.));
#3720=DIRECTION('center_axis',(1.,0.,0.));
#3721=DIRECTION('ref_axis',(0.,0.,-1.));
#3722=DIRECTION('',(0.,1.,0.));
#3723=DIRECTION('center_axis',(-1.,0.,0.));
#3724=DIRECTION('ref_axis',(0.,0.,1.));
#3725=DIRECTION('',(0.,-1.,0.));
#3726=DIRECTION('',(0.,1.,0.));
#3727=DIRECTION('center_axis',(0.,0.,-1.));
#3728=DIRECTION('ref_axis',(-1.,0.,0.));
#3729=DIRECTION('center_axis',(0.,0.,1.));
#3730=DIRECTION('ref_axis',(1.,0.,0.));
#3731=DIRECTION('center_axis',(0.,0.,1.));
#3732=DIRECTION('ref_axis',(1.,0.,0.));
#3733=DIRECTION('',(0.,0.,1.));
#3734=DIRECTION('center_axis',(0.,0.,-1.));
#3735=DIRECTION('ref_axis',(1.,0.,0.));
#3736=DIRECTION('center_axis',(0.,0.,1.));
#3737=DIRECTION('ref_axis',(1.,0.,0.));
#3738=DIRECTION('center_axis',(0.,0.,1.));
#3739=DIRECTION('ref_axis',(1.,0.,0.));
#3740=DIRECTION('',(0.,0.,1.));
#3741=DIRECTION('center_axis',(0.,0.,-1.));
#3742=DIRECTION('ref_axis',(1.,0.,0.));
#3743=DIRECTION('center_axis',(0.,0.,1.));
#3744=DIRECTION('ref_axis',(1.,0.,0.));
#3745=DIRECTION('center_axis',(0.,0.,1.));
#3746=DIRECTION('ref_axis',(1.,0.,0.));
#3747=DIRECTION('',(0.,0.,1.));
#3748=DIRECTION('center_axis',(0.,0.,-1.));
#3749=DIRECTION('ref_axis',(1.,0.,0.));
#3750=DIRECTION('center_axis',(0.,0.,1.));
#3751=DIRECTION('ref_axis',(1.,0.,0.));
#3752=DIRECTION('center_axis',(0.,0.,1.));
#3753=DIRECTION('ref_axis',(1.,0.,0.));
#3754=DIRECTION('',(0.,0.,1.));
#3755=DIRECTION('center_axis',(0.,0.,-1.));
#3756=DIRECTION('ref_axis',(1.,0.,0.));
#3757=DIRECTION('center_axis',(0.,1.,0.));
#3758=DIRECTION('ref_axis',(-1.,0.,0.));
#3759=DIRECTION('',(-1.,0.,0.));
#3760=DIRECTION('',(0.,0.,1.));
#3761=DIRECTION('',(-1.,0.,0.));
#3762=DIRECTION('',(0.,0.,1.));
#3763=DIRECTION('center_axis',(1.,0.,0.));
#3764=DIRECTION('ref_axis',(0.,1.,0.));
#3765=DIRECTION('',(0.,1.,0.));
#3766=DIRECTION('',(0.,1.,0.));
#3767=DIRECTION('',(0.,0.,1.));
#3768=DIRECTION('center_axis',(0.,-1.,0.));
#3769=DIRECTION('ref_axis',(1.,0.,0.));
#3770=DIRECTION('',(1.,0.,0.));
#3771=DIRECTION('',(1.,0.,0.));
#3772=DIRECTION('',(0.,0.,1.));
#3773=DIRECTION('center_axis',(-1.,0.,0.));
#3774=DIRECTION('ref_axis',(0.,-1.,0.));
#3775=DIRECTION('',(0.,-1.,0.));
#3776=DIRECTION('',(0.,-1.,0.));
#3777=DIRECTION('center_axis',(0.,0.,1.));
#3778=DIRECTION('ref_axis',(1.,0.,0.));
#3779=DIRECTION('center_axis',(0.,0.,1.));
#3780=DIRECTION('ref_axis',(1.,0.,0.));
#4497=CARTESIAN_POINT('',(0.,0.,0.));
#4498=CARTESIAN_POINT('Origin',(-4.,0.64,9.9));
#4499=CARTESIAN_POINT('',(-4.,-0.64,10.8));
#4500=CARTESIAN_POINT('',(-4.,0.64,10.8));
#4501=CARTESIAN_POINT('',(-4.,0.32,10.8));
#4502=CARTESIAN_POINT('',(-4.,-0.64,10.));
#4503=CARTESIAN_POINT('',(-4.,-0.64,9.9));
#4504=CARTESIAN_POINT('',(-4.,0.64,10.));
#4505=CARTESIAN_POINT('',(-4.,0.32,10.));
#4506=CARTESIAN_POINT('',(-4.,0.64,9.9));
#4507=CARTESIAN_POINT('Origin',(-4.,-0.64,9.9));
#4508=CARTESIAN_POINT('',(1.2,-0.64,10.8));
#4509=CARTESIAN_POINT('',(-2.,-0.64,10.8));
#4510=CARTESIAN_POINT('',(1.2,-0.64,10.));
#4511=CARTESIAN_POINT('',(1.2,-0.64,9.9));
#4512=CARTESIAN_POINT('',(-2.4,-0.64,10.));
#4513=CARTESIAN_POINT('',(-2.,-0.64,10.));
#4514=CARTESIAN_POINT('',(-2.4,-0.64,9.9));
#4515=CARTESIAN_POINT('',(-2.4,-0.64,10.));
#4516=CARTESIAN_POINT('',(-3.6,-0.64,9.9));
#4517=CARTESIAN_POINT('',(-4.,-0.64,9.9));
#4518=CARTESIAN_POINT('',(-3.6,-0.64,10.));
#4519=CARTESIAN_POINT('',(-3.6,-0.64,9.15));
#4520=CARTESIAN_POINT('',(-2.,-0.64,10.));
#4521=CARTESIAN_POINT('Origin',(-1.4,0.,9.9));
#4522=CARTESIAN_POINT('',(-2.4,-0.62,9.9));
#4523=CARTESIAN_POINT('',(-2.4,-0.51,9.9));
#4524=CARTESIAN_POINT('',(-3.6,-0.62,9.9));
#4525=CARTESIAN_POINT('',(-2.2,-0.62,9.9));
#4526=CARTESIAN_POINT('',(-3.6,-0.51,9.9));
#4527=CARTESIAN_POINT('Origin',(-1.4,0.,9.9));
#4528=CARTESIAN_POINT('',(-2.4,0.64,9.9));
#4529=CARTESIAN_POINT('',(-2.4,0.62,9.9));
#4530=CARTESIAN_POINT('',(-2.4,0.31,9.9));
#4531=CARTESIAN_POINT('',(-3.6,0.64,9.9));
#4532=CARTESIAN_POINT('',(1.2,0.64,9.9));
#4533=CARTESIAN_POINT('',(-3.6,0.62,9.9));
#4534=CARTESIAN_POINT('',(-3.6,0.31,9.9));
#4535=CARTESIAN_POINT('',(-2.2,0.62,9.9));
#4536=CARTESIAN_POINT('Origin',(1.2,0.64,9.9));
#4537=CARTESIAN_POINT('',(1.2,0.64,10.8));
#4538=CARTESIAN_POINT('',(0.6,0.64,10.8));
#4539=CARTESIAN_POINT('',(-3.6,0.64,10.));
#4540=CARTESIAN_POINT('',(0.6,0.64,10.));
#4541=CARTESIAN_POINT('',(-3.6,0.64,9.15));
#4542=CARTESIAN_POINT('',(-2.4,0.64,10.));
#4543=CARTESIAN_POINT('',(-2.4,0.64,10.));
#4544=CARTESIAN_POINT('',(1.2,0.64,10.));
#4545=CARTESIAN_POINT('',(0.6,0.64,10.));
#4546=CARTESIAN_POINT('',(1.2,0.64,9.9));
#4547=CARTESIAN_POINT('Origin',(1.2,-0.64,9.9));
#4548=CARTESIAN_POINT('',(1.2,-0.32,10.8));
#4549=CARTESIAN_POINT('',(1.2,-0.32,10.));
#4550=CARTESIAN_POINT('Origin',(-3.,0.62,9.25));
#4551=CARTESIAN_POINT('',(-3.6,0.62,8.4));
#4552=CARTESIAN_POINT('',(-3.6,0.62,10.1));
#4553=CARTESIAN_POINT('',(-2.4,0.62,8.4));
#4554=CARTESIAN_POINT('',(-3.6,0.62,8.4));
#4555=CARTESIAN_POINT('',(-2.4,0.62,8.4));
#4556=CARTESIAN_POINT('',(-3.325,0.62,9.));
#4557=CARTESIAN_POINT('Origin',(-3.,0.62,9.));
#4558=CARTESIAN_POINT('Origin',(-3.6,0.62,8.4));
#4559=CARTESIAN_POINT('',(-3.6,1.02,10.));
#4560=CARTESIAN_POINT('',(-3.6,0.31,10.));
#4561=CARTESIAN_POINT('',(-3.6,1.02,8.4));
#4562=CARTESIAN_POINT('',(-3.6,1.02,10.1));
#4563=CARTESIAN_POINT('',(-3.6,0.62,8.4));
#4564=CARTESIAN_POINT('Origin',(-3.6,-1.02,8.4));
#4565=CARTESIAN_POINT('',(-3.6,-0.62,8.4));
#4566=CARTESIAN_POINT('',(-3.6,-0.62,10.1));
#4567=CARTESIAN_POINT('',(-3.6,-1.02,8.4));
#4568=CARTESIAN_POINT('',(-3.6,-1.02,8.4));
#4569=CARTESIAN_POINT('',(-3.6,-1.02,10.));
#4570=CARTESIAN_POINT('',(-3.6,-1.02,10.1));
#4571=CARTESIAN_POINT('',(-3.6,-0.51,10.));
#4572=CARTESIAN_POINT('Origin',(-3.,-1.1,9.));
#4573=CARTESIAN_POINT('',(-3.325,-1.02,9.));
#4574=CARTESIAN_POINT('Origin',(-3.,-1.02,9.));
#4575=CARTESIAN_POINT('',(-3.325,-0.62,9.));
#4576=CARTESIAN_POINT('',(-3.325,-1.1,9.));
#4577=CARTESIAN_POINT('Origin',(-3.,-0.62,9.));
#4578=CARTESIAN_POINT('Origin',(-3.,-1.1,9.));
#4579=CARTESIAN_POINT('',(-3.325,1.02,9.));
#4580=CARTESIAN_POINT('',(-3.325,-1.1,9.));
#4581=CARTESIAN_POINT('Origin',(-3.,1.02,9.));
#4582=CARTESIAN_POINT('Origin',(-3.,1.02,9.25));
#4583=CARTESIAN_POINT('',(-2.4,1.02,10.));
#4584=CARTESIAN_POINT('',(-1.5,1.02,10.));
#4585=CARTESIAN_POINT('',(-2.4,1.02,8.4));
#4586=CARTESIAN_POINT('',(-2.4,1.02,8.4));
#4587=CARTESIAN_POINT('',(-3.6,1.02,8.4));
#4588=CARTESIAN_POINT('Origin',(-2.4,0.62,10.1));
#4589=CARTESIAN_POINT('',(-2.4,0.62,8.4));
#4590=CARTESIAN_POINT('',(-2.4,0.31,10.));
#4591=CARTESIAN_POINT('Origin',(-2.4,0.62,8.4));
#4592=CARTESIAN_POINT('Origin',(-3.,-0.62,9.25));
#4593=CARTESIAN_POINT('',(-2.4,-0.62,8.4));
#4594=CARTESIAN_POINT('',(-2.4,-0.62,8.4));
#4595=CARTESIAN_POINT('',(-3.6,-0.62,8.4));
#4596=CARTESIAN_POINT('Origin',(-2.4,-1.02,10.1));
#4597=CARTESIAN_POINT('',(-2.4,-1.02,10.));
#4598=CARTESIAN_POINT('',(-2.4,-0.51,10.));
#4599=CARTESIAN_POINT('',(-2.4,-1.02,8.4));
#4600=CARTESIAN_POINT('',(-2.4,-1.02,8.4));
#4601=CARTESIAN_POINT('',(-2.4,-1.02,8.4));
#4602=CARTESIAN_POINT('Origin',(-2.4,-1.02,8.4));
#4603=CARTESIAN_POINT('',(-3.6,-1.02,8.4));
#4604=CARTESIAN_POINT('Origin',(-3.,-1.02,9.25));
#4605=CARTESIAN_POINT('',(-1.5,-1.02,10.));
#4606=CARTESIAN_POINT('Origin',(0.,-2.1,5.));
#4607=CARTESIAN_POINT('',(0.6,-1.5,5.));
#4608=CARTESIAN_POINT('',(-0.6,-1.5,5.));
#4609=CARTESIAN_POINT('Origin',(0.,-1.5,5.));
#4610=CARTESIAN_POINT('',(0.6,-2.,5.));
#4611=CARTESIAN_POINT('',(0.6,-2.1,5.));
#4612=CARTESIAN_POINT('',(-0.6,-2.,5.));
#4613=CARTESIAN_POINT('Origin',(0.,-2.,5.));
#4614=CARTESIAN_POINT('',(-0.6,-2.1,5.));
#4615=CARTESIAN_POINT('Origin',(0.,-2.1,5.));
#4616=CARTESIAN_POINT('',(0.6,2.,5.));
#4617=CARTESIAN_POINT('',(-0.6,2.,5.));
#4618=CARTESIAN_POINT('Origin',(0.,2.,5.));
#4619=CARTESIAN_POINT('',(0.6,1.5,5.));
#4620=CARTESIAN_POINT('',(0.6,-2.1,5.));
#4621=CARTESIAN_POINT('',(-0.6,1.5,5.));
#4622=CARTESIAN_POINT('Origin',(0.,1.5,5.));
#4623=CARTESIAN_POINT('',(-0.6,-2.1,5.));
#4624=CARTESIAN_POINT('Origin',(0.,1.5,7.55));
#4625=CARTESIAN_POINT('',(1.4,1.5,5.));
#4626=CARTESIAN_POINT('',(-1.4,1.5,5.));
#4627=CARTESIAN_POINT('',(1.4,1.5,10.));
#4628=CARTESIAN_POINT('',(1.4,1.5,5.));
#4629=CARTESIAN_POINT('',(-1.4,1.5,10.));
#4630=CARTESIAN_POINT('',(0.,1.5,10.));
#4631=CARTESIAN_POINT('',(-1.4,1.5,5.));
#4632=CARTESIAN_POINT('',(-1.4,1.5,10.1));
#4633=CARTESIAN_POINT('',(-1.4,1.5,5.));
#4634=CARTESIAN_POINT('Origin',(1.4,1.5,5.));
#4635=CARTESIAN_POINT('',(1.4,2.,5.));
#4636=CARTESIAN_POINT('',(-1.4,2.,5.));
#4637=CARTESIAN_POINT('',(1.4,1.5,5.));
#4638=CARTESIAN_POINT('Origin',(0.,-2.,7.55));
#4639=CARTESIAN_POINT('',(1.4,-2.,5.));
#4640=CARTESIAN_POINT('',(-1.4,-2.,5.));
#4641=CARTESIAN_POINT('',(1.4,-2.,10.));
#4642=CARTESIAN_POINT('',(1.4,-2.,5.));
#4643=CARTESIAN_POINT('',(-1.4,-2.,10.));
#4644=CARTESIAN_POINT('',(0.,-2.,10.));
#4645=CARTESIAN_POINT('',(-1.4,-2.,5.));
#4646=CARTESIAN_POINT('',(-1.4,-2.,10.1));
#4647=CARTESIAN_POINT('',(-1.4,-2.,5.));
#4648=CARTESIAN_POINT('Origin',(1.4,-2.,5.));
#4649=CARTESIAN_POINT('',(1.4,-1.5,5.));
#4650=CARTESIAN_POINT('',(-1.4,-1.5,5.));
#4651=CARTESIAN_POINT('',(1.4,-2.,5.));
#4652=CARTESIAN_POINT('Origin',(0.,2.,7.55));
#4653=CARTESIAN_POINT('',(-1.4,2.,5.));
#4654=CARTESIAN_POINT('',(-1.4,2.,5.));
#4655=CARTESIAN_POINT('',(-1.4,2.,10.));
#4656=CARTESIAN_POINT('',(-1.4,2.,10.1));
#4657=CARTESIAN_POINT('',(1.4,2.,10.));
#4658=CARTESIAN_POINT('',(0.,2.,10.));
#4659=CARTESIAN_POINT('',(1.4,2.,5.));
#4660=CARTESIAN_POINT('Origin',(1.4,1.5,10.1));
#4661=CARTESIAN_POINT('',(1.4,0.75,10.));
#4662=CARTESIAN_POINT('Origin',(-1.4,1.5,5.));
#4663=CARTESIAN_POINT('',(-1.4,0.75,10.));
#4664=CARTESIAN_POINT('',(-1.4,1.5,5.));
#4665=CARTESIAN_POINT('Origin',(1.4,1.5,5.));
#4666=CARTESIAN_POINT('Origin',(0.,-1.5,7.55));
#4667=CARTESIAN_POINT('',(-1.4,-1.5,5.));
#4668=CARTESIAN_POINT('',(-1.4,-1.5,5.));
#4669=CARTESIAN_POINT('',(-1.4,-1.5,10.));
#4670=CARTESIAN_POINT('',(-1.4,-1.5,10.1));
#4671=CARTESIAN_POINT('',(1.4,-1.5,10.));
#4672=CARTESIAN_POINT('',(0.,-1.5,10.));
#4673=CARTESIAN_POINT('',(1.4,-1.5,5.));
#4674=CARTESIAN_POINT('Origin',(1.4,-2.,10.1));
#4675=CARTESIAN_POINT('',(1.4,-1.,10.));
#4676=CARTESIAN_POINT('Origin',(-1.4,-2.,5.));
#4677=CARTESIAN_POINT('',(-1.4,-1.,10.));
#4678=CARTESIAN_POINT('',(-1.4,-2.,5.));
#4679=CARTESIAN_POINT('Origin',(1.4,-2.,5.));
#4680=CARTESIAN_POINT('Origin',(4.,-3.,9.9));
#4681=CARTESIAN_POINT('',(3.575,-3.,10.));
#4682=CARTESIAN_POINT('Origin',(4.,-3.,10.));
#4683=CARTESIAN_POINT('',(3.575,-3.,10.8));
#4684=CARTESIAN_POINT('',(3.575,-3.,9.9));
#4685=CARTESIAN_POINT('Origin',(4.,-3.,10.8));
#4686=CARTESIAN_POINT('Origin',(-4.,3.,9.9));
#4687=CARTESIAN_POINT('',(-4.425,3.,10.));
#4688=CARTESIAN_POINT('Origin',(-4.,3.,10.));
#4689=CARTESIAN_POINT('',(-4.425,3.,10.8));
#4690=CARTESIAN_POINT('',(-4.425,3.,9.9));
#4691=CARTESIAN_POINT('Origin',(-4.,3.,10.8));
#4692=CARTESIAN_POINT('Origin',(-4.,-3.,9.9));
#4693=CARTESIAN_POINT('',(-4.425,-3.,10.));
#4694=CARTESIAN_POINT('Origin',(-4.,-3.,10.));
#4695=CARTESIAN_POINT('',(-4.425,-3.,10.8));
#4696=CARTESIAN_POINT('',(-4.425,-3.,9.9));
#4697=CARTESIAN_POINT('Origin',(-4.,-3.,10.8));
#4698=CARTESIAN_POINT('Origin',(4.,3.,9.9));
#4699=CARTESIAN_POINT('',(3.575,3.,10.));
#4700=CARTESIAN_POINT('Origin',(4.,3.,10.));
#4701=CARTESIAN_POINT('',(3.575,3.,10.8));
#4702=CARTESIAN_POINT('',(3.575,3.,9.9));
#4703=CARTESIAN_POINT('Origin',(4.,3.,10.8));
#4704=CARTESIAN_POINT('Origin',(5.,4.,10.));
#4705=CARTESIAN_POINT('',(5.,4.,10.));
#4706=CARTESIAN_POINT('',(-5.,4.,10.));
#4707=CARTESIAN_POINT('',(5.,4.,10.));
#4708=CARTESIAN_POINT('',(-5.,4.,10.8));
#4709=CARTESIAN_POINT('',(-5.,4.,10.));
#4710=CARTESIAN_POINT('',(5.,4.,10.8));
#4711=CARTESIAN_POINT('',(5.,4.,10.8));
#4712=CARTESIAN_POINT('',(5.,4.,10.));
#4713=CARTESIAN_POINT('Origin',(5.,-4.,10.));
#4714=CARTESIAN_POINT('',(5.,-4.,10.));
#4715=CARTESIAN_POINT('',(5.,-4.,10.));
#4716=CARTESIAN_POINT('',(5.,-4.,10.8));
#4717=CARTESIAN_POINT('',(5.,-4.,10.8));
#4718=CARTESIAN_POINT('',(5.,-4.,10.));
#4719=CARTESIAN_POINT('Origin',(-5.,-4.,10.));
#4720=CARTESIAN_POINT('',(-5.,-4.,10.));
#4721=CARTESIAN_POINT('',(-5.,-4.,10.));
#4722=CARTESIAN_POINT('',(-5.,-4.,10.8));
#4723=CARTESIAN_POINT('',(-5.,-4.,10.8));
#4724=CARTESIAN_POINT('',(-5.,-4.,10.));
#4725=CARTESIAN_POINT('Origin',(-5.,4.,10.));
#4726=CARTESIAN_POINT('',(-5.,4.,10.));
#4727=CARTESIAN_POINT('',(-5.,4.,10.8));
#4728=CARTESIAN_POINT('Origin',(0.,0.,10.8));
#4729=CARTESIAN_POINT('Origin',(0.,0.,10.));
#5691=UNCERTAINTY_MEASURE_WITH_UNIT(LENGTH_MEASURE(0.001),#5735,
'DISTANCE_ACCURACY_VALUE',
'Maximum model space distance between geometric entities at asserted c
onnectivities');
#5711=UNCERTAINTY_MEASURE_WITH_UNIT(LENGTH_MEASURE(0.001),#5735,
'DISTANCE_ACCURACY_VALUE',
'Maximum model space distance between geometric entities at asserted c
onnectivities');
#5714=(
GEOMETRIC_REPRESENTATION_CONTEXT(3)
GLOBAL_UNCERTAINTY_ASSIGNED_CONTEXT((#5691))
GLOBAL_UNIT_ASSIGNED_CONTEXT((#5735,#5737,#5738))
REPRESENTATION_CONTEXT('','3D')
);
#5734=(
GEOMETRIC_REPRESENTATION_CONTEXT(3)
GLOBAL_UNCERTAINTY_ASSIGNED_CONTEXT((#5711))
GLOBAL_UNIT_ASSIGNED_CONTEXT((#5735,#5737,#5738))
REPRESENTATION_CONTEXT('','3D')
);
#5735=(
LENGTH_UNIT()
NAMED_UNIT(*)
SI_UNIT(.CENTI.,.METRE.)
);
#5737=(
NAMED_UNIT(*)
PLANE_ANGLE_UNIT()
SI_UNIT($,.RADIAN.)
);
#5738=(
NAMED_UNIT(*)
SI_UNIT($,.STERADIAN.)
SOLID_ANGLE_UNIT()
);
#5741=SHAPE_DEFINITION_REPRESENTATION(#5763,#5810);
#5763=PRODUCT_DEFINITION_SHAPE('',$,#5833);
#5810=SHAPE_REPRESENTATION('',(#3202),#5714);
#5830=PRODUCT_DEFINITION_CONTEXT('part definition',#5898,'design');
#5833=PRODUCT_DEFINITION('Fixed fork with pedal bearings',
'Fixed fork with pedal bearings',#5855,#5830);
#5855=PRODUCT_DEFINITION_FORMATION('',$,#5902);
#5898=APPLICATION_CONTEXT(
'Core Data for Automotive Mechanical Design Process');
#5899=PRODUCT_CONTEXT('part definition',#5898,'mechanical');
#5902=PRODUCT('Fixed fork with pedal bearings',
'Fixed fork with pedal bearings','Fixed fork with pedal bearings',(#5899));
#5978=COLOUR_RGB('Grey',0.48,0.52,0.57);
#5979=FILL_AREA_STYLE_COLOUR('',#5978);
#5980=FILL_AREA_STYLE('',(#5979));
#5981=SURFACE_STYLE_FILL_AREA(#5980);
#5982=SURFACE_SIDE_STYLE('',(#5981));
#5983=SURFACE_STYLE_USAGE(.BOTH.,#5982);
#5984=PRESENTATION_STYLE_ASSIGNMENT((#5983));
ENDSEC;
END-ISO-10303-21;
